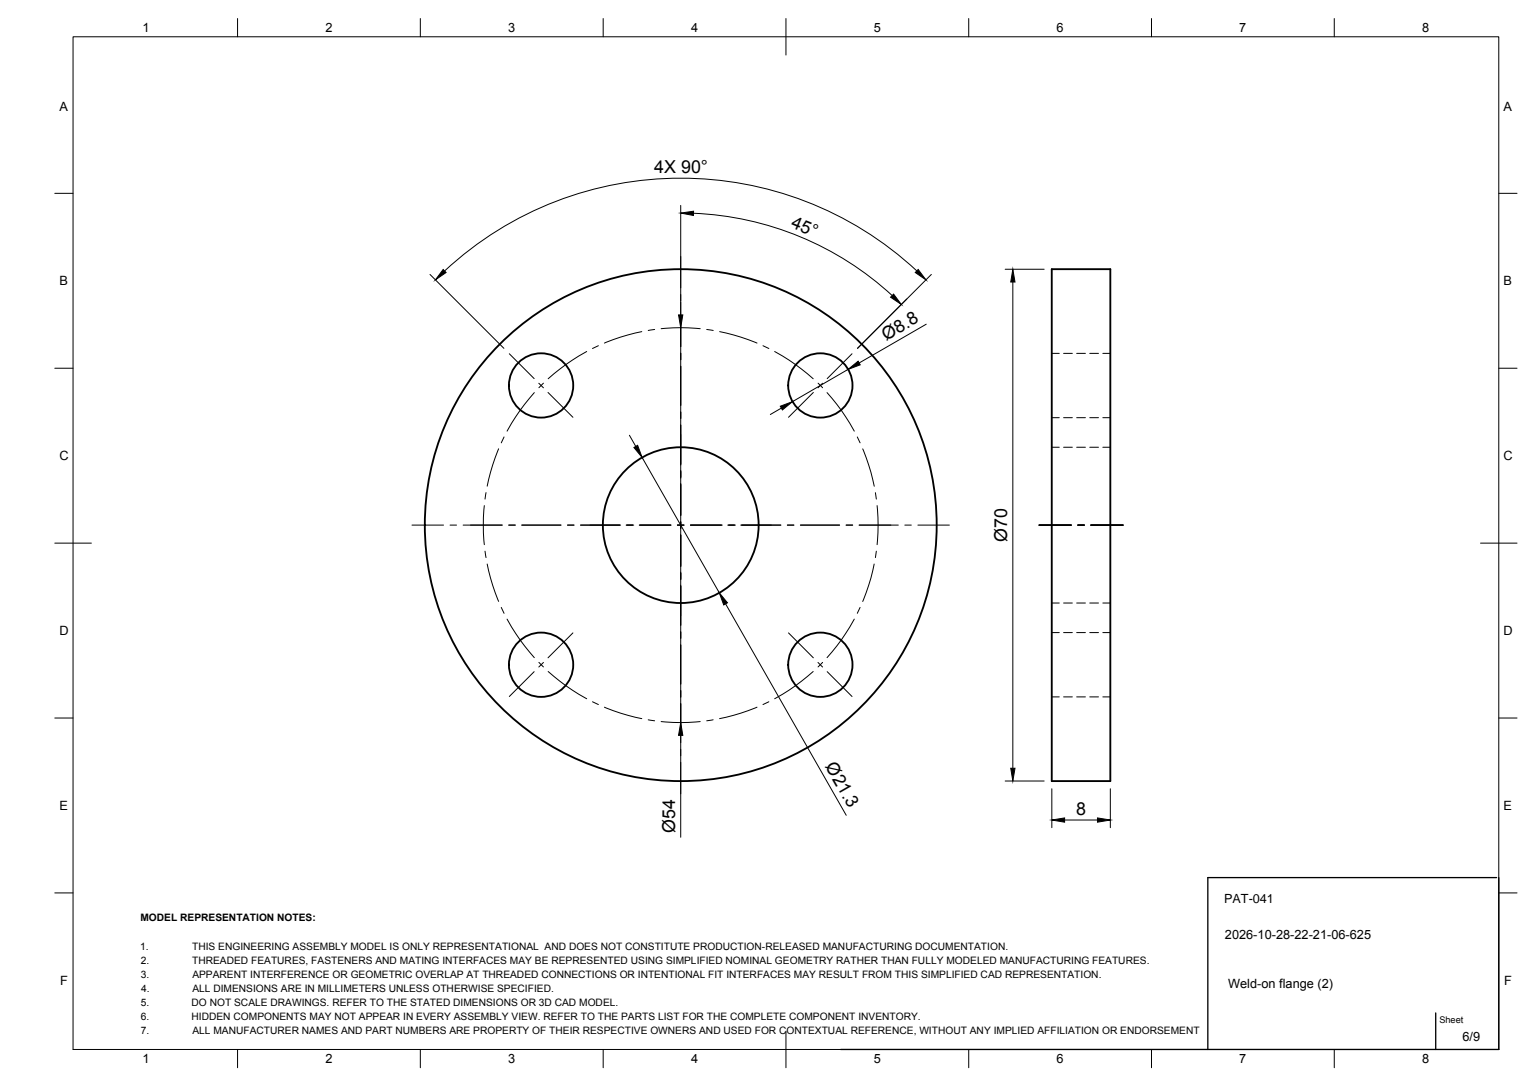
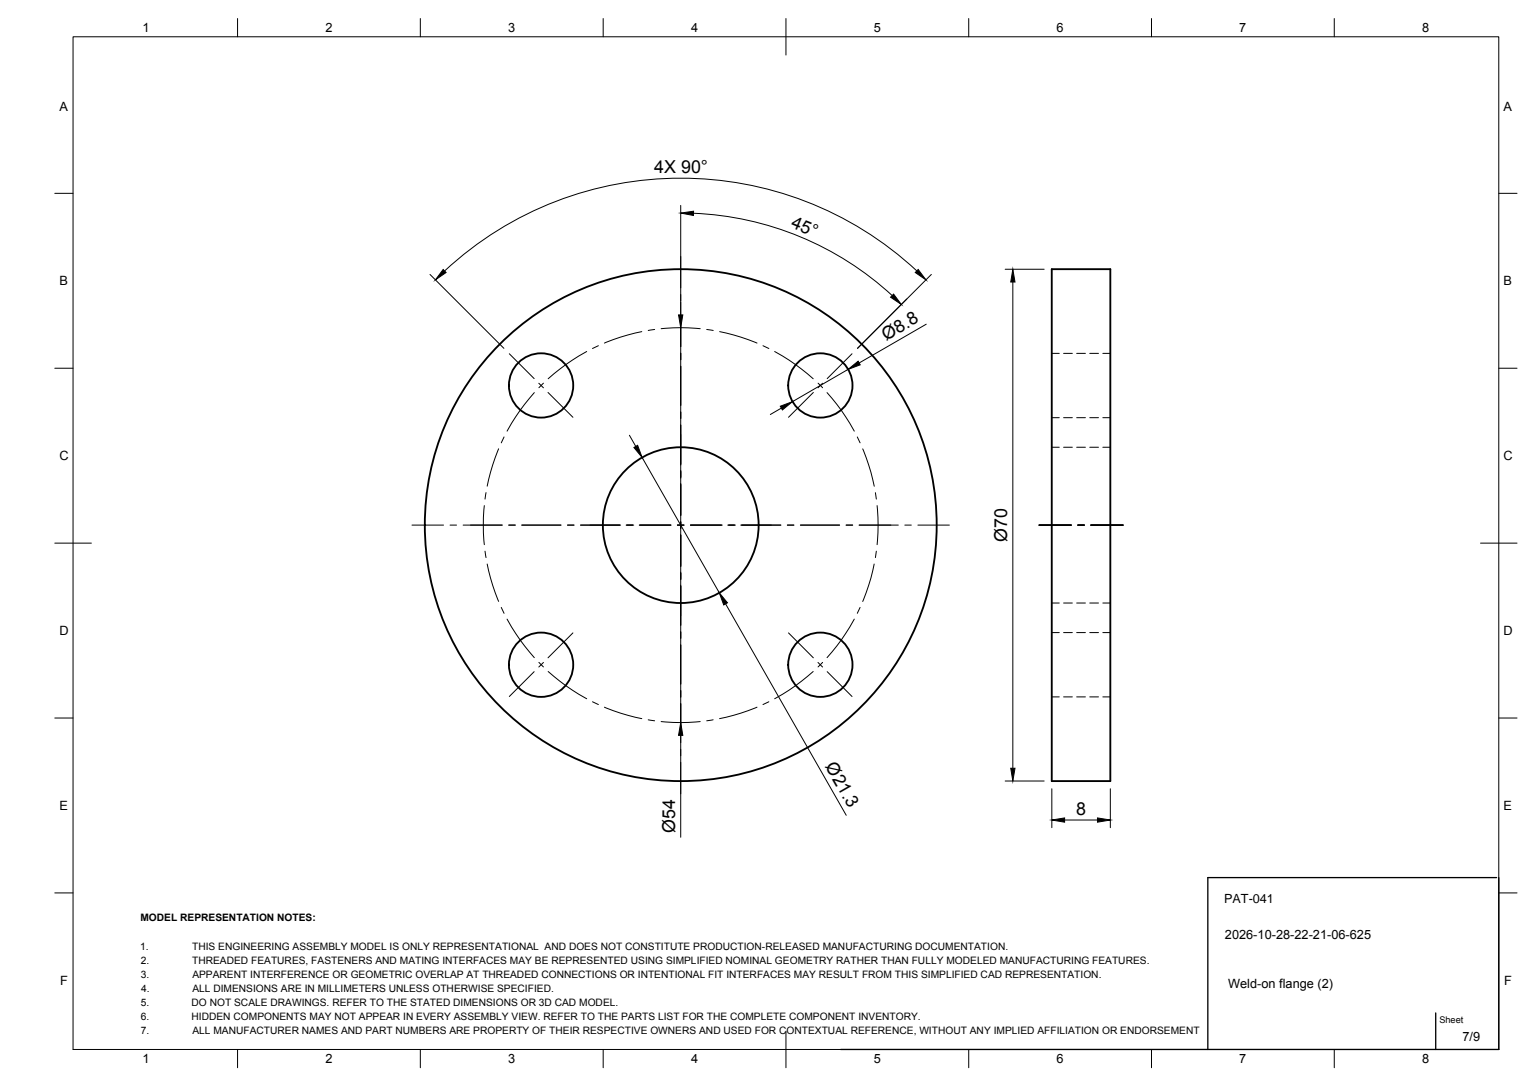
ISO-10303-21;
HEADER;
/* Generated by software containing ST-Developer
 * from STEP Tools, Inc. (www.steptools.com) 
 */

FILE_DESCRIPTION(
/* description */ ('PAT-041'),
/* implementation_level */ '2;1');

FILE_NAME(
/* name */ 'Weld-on flange (2).step',
/* time_stamp */ '2026-10-28T22:21:24-07:00',
/* author */ (''),
/* organization */ (''),
/* preprocessor_version */ 'ST-DEVELOPER v20.2',
/* originating_system */ 'Autodesk Translation Framework v15.17.0.0',
/* authorisation */ '');

FILE_SCHEMA (('AUTOMOTIVE_DESIGN { 1 0 10303 214 3 1 1 }'));
ENDSEC;

DATA;
#10=MECHANICAL_DESIGN_GEOMETRIC_PRESENTATION_REPRESENTATION('',(#212),#2507);
#192=SHAPE_REPRESENTATION_RELATIONSHIP('SRR','None',#2577,#202);
#202=ADVANCED_BREP_SHAPE_REPRESENTATION('',(#222),#2500);
#212=STYLED_ITEM('',(#2687),#222);
#222=MANIFOLD_SOLID_BREP('Body1',#1332);
#251=FACE_BOUND('',#433,.T.);
#252=FACE_BOUND('',#434,.T.);
#253=FACE_BOUND('',#435,.T.);
#254=FACE_BOUND('',#436,.T.);
#255=FACE_BOUND('',#437,.T.);
#256=FACE_BOUND('',#439,.T.);
#257=FACE_BOUND('',#440,.T.);
#258=FACE_BOUND('',#441,.T.);
#259=FACE_BOUND('',#442,.T.);
#260=FACE_BOUND('',#443,.T.);
#286=PLANE('',#1521);
#287=PLANE('',#1522);
#333=FACE_OUTER_BOUND('',#426,.T.);
#334=FACE_OUTER_BOUND('',#427,.T.);
#335=FACE_OUTER_BOUND('',#428,.T.);
#336=FACE_OUTER_BOUND('',#429,.T.);
#337=FACE_OUTER_BOUND('',#430,.T.);
#338=FACE_OUTER_BOUND('',#431,.T.);
#339=FACE_OUTER_BOUND('',#432,.T.);
#340=FACE_OUTER_BOUND('',#438,.T.);
#426=EDGE_LOOP('',(#1016,#1017,#1018,#1019));
#427=EDGE_LOOP('',(#1020,#1021,#1022,#1023));
#428=EDGE_LOOP('',(#1024,#1025,#1026,#1027));
#429=EDGE_LOOP('',(#1028,#1029,#1030,#1031));
#430=EDGE_LOOP('',(#1032,#1033,#1034,#1035));
#431=EDGE_LOOP('',(#1036,#1037,#1038,#1039));
#432=EDGE_LOOP('',(#1040));
#433=EDGE_LOOP('',(#1041));
#434=EDGE_LOOP('',(#1042));
#435=EDGE_LOOP('',(#1043));
#436=EDGE_LOOP('',(#1044));
#437=EDGE_LOOP('',(#1045));
#438=EDGE_LOOP('',(#1046));
#439=EDGE_LOOP('',(#1047));
#440=EDGE_LOOP('',(#1048));
#441=EDGE_LOOP('',(#1049));
#442=EDGE_LOOP('',(#1050));
#443=EDGE_LOOP('',(#1051));
#520=LINE('',#2184,#576);
#521=LINE('',#2190,#577);
#522=LINE('',#2196,#578);
#523=LINE('',#2202,#579);
#524=LINE('',#2208,#580);
#525=LINE('',#2214,#581);
#576=VECTOR('',#1767,0.44);
#577=VECTOR('',#1774,0.44);
#578=VECTOR('',#1781,0.44);
#579=VECTOR('',#1788,0.44);
#580=VECTOR('',#1795,1.065);
#581=VECTOR('',#1802,3.5);
#646=CIRCLE('',#1504,0.44);
#647=CIRCLE('',#1505,0.44);
#648=CIRCLE('',#1507,0.44);
#649=CIRCLE('',#1508,0.44);
#650=CIRCLE('',#1510,0.44);
#651=CIRCLE('',#1511,0.44);
#652=CIRCLE('',#1513,0.44);
#653=CIRCLE('',#1514,0.44);
#654=CIRCLE('',#1516,1.065);
#655=CIRCLE('',#1517,1.065);
#656=CIRCLE('',#1519,3.5);
#657=CIRCLE('',#1520,3.5);
#718=VERTEX_POINT('',#2181);
#719=VERTEX_POINT('',#2183);
#720=VERTEX_POINT('',#2187);
#721=VERTEX_POINT('',#2189);
#722=VERTEX_POINT('',#2193);
#723=VERTEX_POINT('',#2195);
#724=VERTEX_POINT('',#2199);
#725=VERTEX_POINT('',#2201);
#726=VERTEX_POINT('',#2205);
#727=VERTEX_POINT('',#2207);
#728=VERTEX_POINT('',#2211);
#729=VERTEX_POINT('',#2213);
#828=EDGE_CURVE('',#718,#718,#646,.T.);
#829=EDGE_CURVE('',#718,#719,#520,.T.);
#830=EDGE_CURVE('',#719,#719,#647,.T.);
#831=EDGE_CURVE('',#720,#720,#648,.T.);
#832=EDGE_CURVE('',#720,#721,#521,.T.);
#833=EDGE_CURVE('',#721,#721,#649,.T.);
#834=EDGE_CURVE('',#722,#722,#650,.T.);
#835=EDGE_CURVE('',#722,#723,#522,.T.);
#836=EDGE_CURVE('',#723,#723,#651,.T.);
#837=EDGE_CURVE('',#724,#724,#652,.T.);
#838=EDGE_CURVE('',#724,#725,#523,.T.);
#839=EDGE_CURVE('',#725,#725,#653,.T.);
#840=EDGE_CURVE('',#726,#726,#654,.T.);
#841=EDGE_CURVE('',#726,#727,#524,.T.);
#842=EDGE_CURVE('',#727,#727,#655,.T.);
#843=EDGE_CURVE('',#728,#728,#656,.T.);
#844=EDGE_CURVE('',#728,#729,#525,.T.);
#845=EDGE_CURVE('',#729,#729,#657,.T.);
#1016=ORIENTED_EDGE('',*,*,#828,.F.);
#1017=ORIENTED_EDGE('',*,*,#829,.T.);
#1018=ORIENTED_EDGE('',*,*,#830,.F.);
#1019=ORIENTED_EDGE('',*,*,#829,.F.);
#1020=ORIENTED_EDGE('',*,*,#831,.F.);
#1021=ORIENTED_EDGE('',*,*,#832,.T.);
#1022=ORIENTED_EDGE('',*,*,#833,.F.);
#1023=ORIENTED_EDGE('',*,*,#832,.F.);
#1024=ORIENTED_EDGE('',*,*,#834,.F.);
#1025=ORIENTED_EDGE('',*,*,#835,.T.);
#1026=ORIENTED_EDGE('',*,*,#836,.F.);
#1027=ORIENTED_EDGE('',*,*,#835,.F.);
#1028=ORIENTED_EDGE('',*,*,#837,.F.);
#1029=ORIENTED_EDGE('',*,*,#838,.T.);
#1030=ORIENTED_EDGE('',*,*,#839,.F.);
#1031=ORIENTED_EDGE('',*,*,#838,.F.);
#1032=ORIENTED_EDGE('',*,*,#840,.F.);
#1033=ORIENTED_EDGE('',*,*,#841,.T.);
#1034=ORIENTED_EDGE('',*,*,#842,.T.);
#1035=ORIENTED_EDGE('',*,*,#841,.F.);
#1036=ORIENTED_EDGE('',*,*,#843,.F.);
#1037=ORIENTED_EDGE('',*,*,#844,.T.);
#1038=ORIENTED_EDGE('',*,*,#845,.T.);
#1039=ORIENTED_EDGE('',*,*,#844,.F.);
#1040=ORIENTED_EDGE('',*,*,#843,.T.);
#1041=ORIENTED_EDGE('',*,*,#840,.T.);
#1042=ORIENTED_EDGE('',*,*,#839,.T.);
#1043=ORIENTED_EDGE('',*,*,#836,.T.);
#1044=ORIENTED_EDGE('',*,*,#833,.T.);
#1045=ORIENTED_EDGE('',*,*,#830,.T.);
#1046=ORIENTED_EDGE('',*,*,#845,.F.);
#1047=ORIENTED_EDGE('',*,*,#842,.F.);
#1048=ORIENTED_EDGE('',*,*,#837,.T.);
#1049=ORIENTED_EDGE('',*,*,#834,.T.);
#1050=ORIENTED_EDGE('',*,*,#831,.T.);
#1051=ORIENTED_EDGE('',*,*,#828,.T.);
#1238=CYLINDRICAL_SURFACE('',#1503,0.44);
#1239=CYLINDRICAL_SURFACE('',#1506,0.44);
#1240=CYLINDRICAL_SURFACE('',#1509,0.44);
#1241=CYLINDRICAL_SURFACE('',#1512,0.44);
#1242=CYLINDRICAL_SURFACE('',#1515,1.065);
#1243=CYLINDRICAL_SURFACE('',#1518,3.5);
#1278=ADVANCED_FACE('',(#333),#1238,.F.);
#1279=ADVANCED_FACE('',(#334),#1239,.F.);
#1280=ADVANCED_FACE('',(#335),#1240,.F.);
#1281=ADVANCED_FACE('',(#336),#1241,.F.);
#1282=ADVANCED_FACE('',(#337),#1242,.F.);
#1283=ADVANCED_FACE('',(#338),#1243,.T.);
#1284=ADVANCED_FACE('',(#339,#251,#252,#253,#254,#255),#286,.T.);
#1285=ADVANCED_FACE('',(#340,#256,#257,#258,#259,#260),#287,.F.);
#1332=CLOSED_SHELL('',(#1278,#1279,#1280,#1281,#1282,#1283,#1284,#1285));
#1502=AXIS2_PLACEMENT_3D('',#2179,#1761,#1762);
#1503=AXIS2_PLACEMENT_3D('',#2180,#1763,#1764);
#1504=AXIS2_PLACEMENT_3D('',#2182,#1765,#1766);
#1505=AXIS2_PLACEMENT_3D('',#2185,#1768,#1769);
#1506=AXIS2_PLACEMENT_3D('',#2186,#1770,#1771);
#1507=AXIS2_PLACEMENT_3D('',#2188,#1772,#1773);
#1508=AXIS2_PLACEMENT_3D('',#2191,#1775,#1776);
#1509=AXIS2_PLACEMENT_3D('',#2192,#1777,#1778);
#1510=AXIS2_PLACEMENT_3D('',#2194,#1779,#1780);
#1511=AXIS2_PLACEMENT_3D('',#2197,#1782,#1783);
#1512=AXIS2_PLACEMENT_3D('',#2198,#1784,#1785);
#1513=AXIS2_PLACEMENT_3D('',#2200,#1786,#1787);
#1514=AXIS2_PLACEMENT_3D('',#2203,#1789,#1790);
#1515=AXIS2_PLACEMENT_3D('',#2204,#1791,#1792);
#1516=AXIS2_PLACEMENT_3D('',#2206,#1793,#1794);
#1517=AXIS2_PLACEMENT_3D('',#2209,#1796,#1797);
#1518=AXIS2_PLACEMENT_3D('',#2210,#1798,#1799);
#1519=AXIS2_PLACEMENT_3D('',#2212,#1800,#1801);
#1520=AXIS2_PLACEMENT_3D('',#2215,#1803,#1804);
#1521=AXIS2_PLACEMENT_3D('',#2216,#1805,#1806);
#1522=AXIS2_PLACEMENT_3D('',#2217,#1807,#1808);
#1761=DIRECTION('axis',(0.,0.,1.));
#1762=DIRECTION('refdir',(1.,0.,0.));
#1763=DIRECTION('center_axis',(1.,0.,0.));
#1764=DIRECTION('ref_axis',(0.,0.,-1.));
#1765=DIRECTION('center_axis',(1.,0.,0.));
#1766=DIRECTION('ref_axis',(0.,0.,-1.));
#1767=DIRECTION('',(1.,0.,0.));
#1768=DIRECTION('center_axis',(-1.,0.,0.));
#1769=DIRECTION('ref_axis',(0.,0.,-1.));
#1770=DIRECTION('center_axis',(1.,0.,0.));
#1771=DIRECTION('ref_axis',(0.,0.,-1.));
#1772=DIRECTION('center_axis',(1.,0.,0.));
#1773=DIRECTION('ref_axis',(0.,0.,-1.));
#1774=DIRECTION('',(1.,0.,0.));
#1775=DIRECTION('center_axis',(-1.,0.,0.));
#1776=DIRECTION('ref_axis',(0.,0.,-1.));
#1777=DIRECTION('center_axis',(1.,0.,0.));
#1778=DIRECTION('ref_axis',(0.,0.,-1.));
#1779=DIRECTION('center_axis',(1.,0.,0.));
#1780=DIRECTION('ref_axis',(0.,0.,-1.));
#1781=DIRECTION('',(1.,0.,0.));
#1782=DIRECTION('center_axis',(-1.,0.,0.));
#1783=DIRECTION('ref_axis',(0.,0.,-1.));
#1784=DIRECTION('center_axis',(1.,0.,0.));
#1785=DIRECTION('ref_axis',(0.,0.,-1.));
#1786=DIRECTION('center_axis',(1.,0.,0.));
#1787=DIRECTION('ref_axis',(0.,0.,-1.));
#1788=DIRECTION('',(1.,0.,0.));
#1789=DIRECTION('center_axis',(-1.,0.,0.));
#1790=DIRECTION('ref_axis',(0.,0.,-1.));
#1791=DIRECTION('center_axis',(1.,0.,0.));
#1792=DIRECTION('ref_axis',(0.,0.,-1.));
#1793=DIRECTION('center_axis',(-1.,0.,0.));
#1794=DIRECTION('ref_axis',(0.,0.,-1.));
#1795=DIRECTION('',(-1.,0.,0.));
#1796=DIRECTION('center_axis',(-1.,0.,0.));
#1797=DIRECTION('ref_axis',(0.,0.,-1.));
#1798=DIRECTION('center_axis',(1.,0.,0.));
#1799=DIRECTION('ref_axis',(0.,0.,-1.));
#1800=DIRECTION('center_axis',(1.,0.,0.));
#1801=DIRECTION('ref_axis',(0.,0.,-1.));
#1802=DIRECTION('',(-1.,0.,0.));
#1803=DIRECTION('center_axis',(1.,0.,0.));
#1804=DIRECTION('ref_axis',(0.,0.,-1.));
#1805=DIRECTION('center_axis',(1.,0.,0.));
#1806=DIRECTION('ref_axis',(0.,0.,-1.));
#1807=DIRECTION('center_axis',(1.,0.,0.));
#1808=DIRECTION('ref_axis',(0.,0.,-1.));
#2179=CARTESIAN_POINT('',(0.,0.,0.));
#2180=CARTESIAN_POINT('Origin',(-11.1,-1.90918830920368,-1.90918830920368));
#2181=CARTESIAN_POINT('',(-11.,-1.90918830920368,-1.46918830920368));
#2182=CARTESIAN_POINT('Origin',(-11.,-1.90918830920368,-1.90918830920368));
#2183=CARTESIAN_POINT('',(-10.2,-1.90918830920368,-1.46918830920368));
#2184=CARTESIAN_POINT('',(-11.1,-1.90918830920368,-1.46918830920368));
#2185=CARTESIAN_POINT('Origin',(-10.2,-1.90918830920368,-1.90918830920368));
#2186=CARTESIAN_POINT('Origin',(-11.1,-1.90918830920368,1.90918830920368));
#2187=CARTESIAN_POINT('',(-11.,-1.90918830920368,2.34918830920368));
#2188=CARTESIAN_POINT('Origin',(-11.,-1.90918830920368,1.90918830920368));
#2189=CARTESIAN_POINT('',(-10.2,-1.90918830920368,2.34918830920368));
#2190=CARTESIAN_POINT('',(-11.1,-1.90918830920368,2.34918830920368));
#2191=CARTESIAN_POINT('Origin',(-10.2,-1.90918830920368,1.90918830920368));
#2192=CARTESIAN_POINT('Origin',(-11.1,1.90918830920368,1.90918830920368));
#2193=CARTESIAN_POINT('',(-11.,1.90918830920368,2.34918830920368));
#2194=CARTESIAN_POINT('Origin',(-11.,1.90918830920368,1.90918830920368));
#2195=CARTESIAN_POINT('',(-10.2,1.90918830920368,2.34918830920368));
#2196=CARTESIAN_POINT('',(-11.1,1.90918830920368,2.34918830920368));
#2197=CARTESIAN_POINT('Origin',(-10.2,1.90918830920368,1.90918830920368));
#2198=CARTESIAN_POINT('Origin',(-11.1,1.90918830920368,-1.90918830920368));
#2199=CARTESIAN_POINT('',(-11.,1.90918830920368,-1.46918830920368));
#2200=CARTESIAN_POINT('Origin',(-11.,1.90918830920368,-1.90918830920368));
#2201=CARTESIAN_POINT('',(-10.2,1.90918830920368,-1.46918830920368));
#2202=CARTESIAN_POINT('',(-11.1,1.90918830920368,-1.46918830920368));
#2203=CARTESIAN_POINT('Origin',(-10.2,1.90918830920368,-1.90918830920368));
#2204=CARTESIAN_POINT('Origin',(-11.,0.,0.));
#2205=CARTESIAN_POINT('',(-10.2,-1.30424884109193E-16,1.065));
#2206=CARTESIAN_POINT('Origin',(-10.2,0.,0.));
#2207=CARTESIAN_POINT('',(-11.,-1.30424884109193E-16,1.065));
#2208=CARTESIAN_POINT('',(-11.,-1.30424884109193E-16,1.065));
#2209=CARTESIAN_POINT('Origin',(-11.,0.,0.));
#2210=CARTESIAN_POINT('Origin',(-11.,0.,0.));
#2211=CARTESIAN_POINT('',(-10.2,-4.28626379701574E-16,3.5));
#2212=CARTESIAN_POINT('Origin',(-10.2,0.,0.));
#2213=CARTESIAN_POINT('',(-11.,-4.28626379701574E-16,3.5));
#2214=CARTESIAN_POINT('',(-11.,-4.28626379701574E-16,3.5));
#2215=CARTESIAN_POINT('Origin',(-11.,0.,0.));
#2216=CARTESIAN_POINT('Origin',(-10.2,0.,0.));
#2217=CARTESIAN_POINT('Origin',(-11.,0.,0.));
#2488=UNCERTAINTY_MEASURE_WITH_UNIT(LENGTH_MEASURE(0.001),#2508,
'DISTANCE_ACCURACY_VALUE',
'Maximum model space distance between geometric entities at asserted c
onnectivities');
#2495=UNCERTAINTY_MEASURE_WITH_UNIT(LENGTH_MEASURE(0.001),#2508,
'DISTANCE_ACCURACY_VALUE',
'Maximum model space distance between geometric entities at asserted c
onnectivities');
#2500=(
GEOMETRIC_REPRESENTATION_CONTEXT(3)
GLOBAL_UNCERTAINTY_ASSIGNED_CONTEXT((#2488))
GLOBAL_UNIT_ASSIGNED_CONTEXT((#2508,#2510,#2511))
REPRESENTATION_CONTEXT('','3D')
);
#2507=(
GEOMETRIC_REPRESENTATION_CONTEXT(3)
GLOBAL_UNCERTAINTY_ASSIGNED_CONTEXT((#2495))
GLOBAL_UNIT_ASSIGNED_CONTEXT((#2508,#2510,#2511))
REPRESENTATION_CONTEXT('','3D')
);
#2508=(
LENGTH_UNIT()
NAMED_UNIT(*)
SI_UNIT(.CENTI.,.METRE.)
);
#2510=(
NAMED_UNIT(*)
PLANE_ANGLE_UNIT()
SI_UNIT($,.RADIAN.)
);
#2511=(
NAMED_UNIT(*)
SI_UNIT($,.STERADIAN.)
SOLID_ANGLE_UNIT()
);
#2516=SHAPE_DEFINITION_REPRESENTATION(#2527,#2577);
#2527=PRODUCT_DEFINITION_SHAPE('',$,#2589);
#2577=SHAPE_REPRESENTATION('',(#1502),#2500);
#2584=PRODUCT_DEFINITION_CONTEXT('part definition',#2619,'design');
#2589=PRODUCT_DEFINITION('Weld-on flange (2)','Weld-on flange (2)',
#2600,#2584);
#2600=PRODUCT_DEFINITION_FORMATION('',$,#2625);
#2619=APPLICATION_CONTEXT(
'Core Data for Automotive Mechanical Design Process');
#2620=PRODUCT_CONTEXT('part definition',#2619,'mechanical');
#2625=PRODUCT('Weld-on flange (2)','Weld-on flange (2)',
'Weld-on flange (2)',(#2620));
#2681=COLOUR_RGB('Sky Blue',0.24,0.69,0.87);
#2682=FILL_AREA_STYLE_COLOUR('',#2681);
#2683=FILL_AREA_STYLE('',(#2682));
#2684=SURFACE_STYLE_FILL_AREA(#2683);
#2685=SURFACE_SIDE_STYLE('',(#2684));
#2686=SURFACE_STYLE_USAGE(.BOTH.,#2685);
#2687=PRESENTATION_STYLE_ASSIGNMENT((#2686));
ENDSEC;
END-ISO-10303-21;
